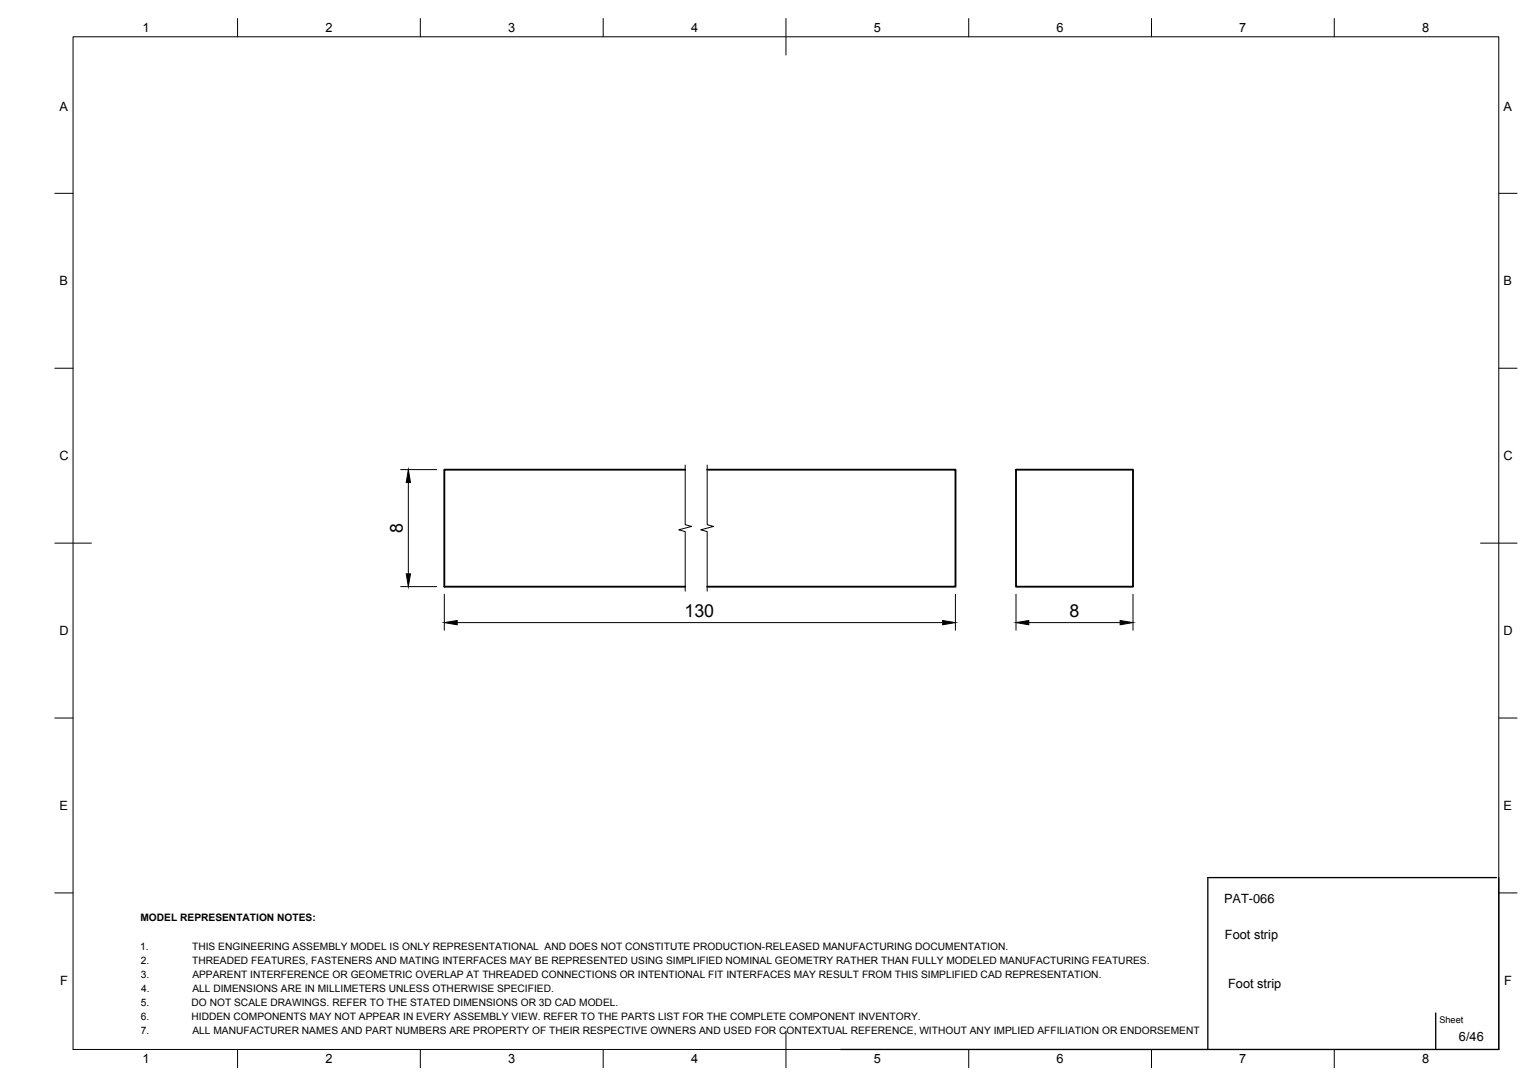
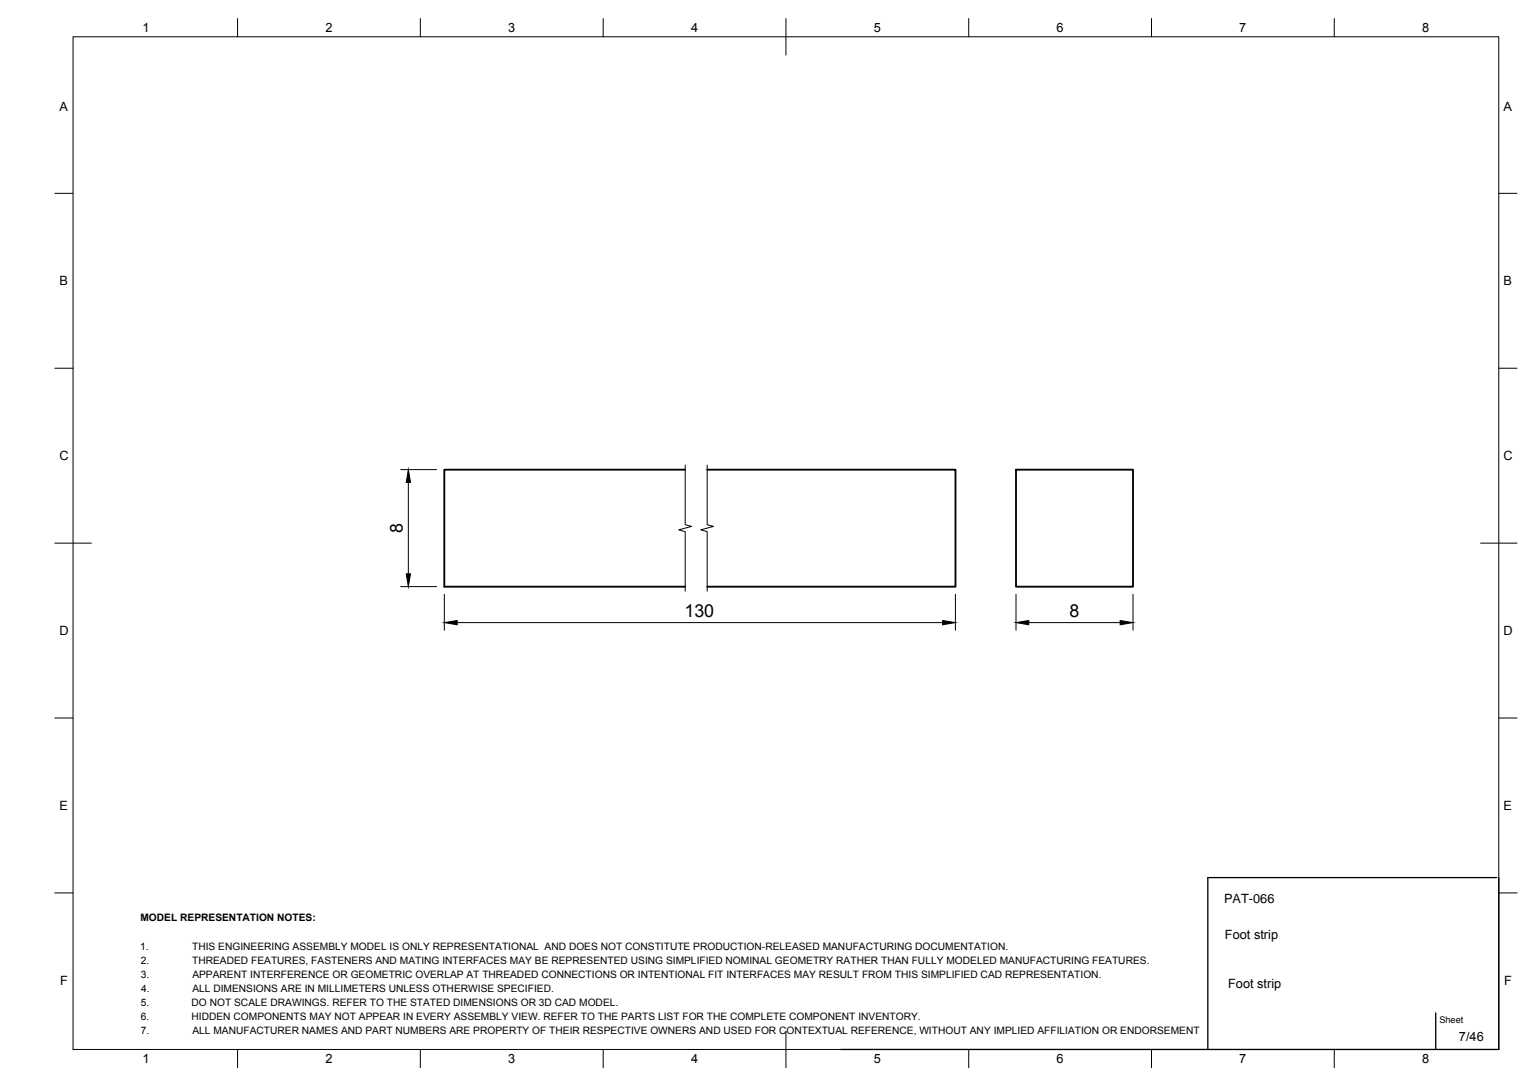
ISO-10303-21;
HEADER;
/* Generated by software containing ST-Developer
 * from STEP Tools, Inc. (www.steptools.com) 
 */

FILE_DESCRIPTION(
/* description */ ('Lever-operated bar clamp (toggle)'),
/* implementation_level */ '2;1');

FILE_NAME(
/* name */ 'Foot strip.step',
/* time_stamp */ '2026-10-28T03:25:02-07:00',
/* author */ (''),
/* organization */ (''),
/* preprocessor_version */ 'ST-DEVELOPER v20.2',
/* originating_system */ 'Autodesk Translation Framework v15.17.0.0',
/* authorisation */ '');

FILE_SCHEMA (('AUTOMOTIVE_DESIGN { 1 0 10303 214 3 1 1 }'));
ENDSEC;

DATA;
#10=MECHANICAL_DESIGN_GEOMETRIC_PRESENTATION_REPRESENTATION('',(#411),#12413);
#335=SHAPE_REPRESENTATION_RELATIONSHIP('SRR','None',#12574,#373);
#373=ADVANCED_BREP_SHAPE_REPRESENTATION('',(#458),#12371);
#411=STYLED_ITEM('',(#12855),#458);
#458=MANIFOLD_SOLID_BREP('Body1',#6570);
#657=PLANE('',#7073);
#658=PLANE('',#7074);
#659=PLANE('',#7075);
#660=PLANE('',#7076);
#661=PLANE('',#7077);
#662=PLANE('',#7078);
#902=FACE_OUTER_BOUND('',#1324,.T.);
#903=FACE_OUTER_BOUND('',#1325,.T.);
#904=FACE_OUTER_BOUND('',#1326,.T.);
#905=FACE_OUTER_BOUND('',#1327,.T.);
#906=FACE_OUTER_BOUND('',#1328,.T.);
#907=FACE_OUTER_BOUND('',#1329,.T.);
#1324=EDGE_LOOP('',(#4493,#4494,#4495,#4496));
#1325=EDGE_LOOP('',(#4497,#4498,#4499,#4500));
#1326=EDGE_LOOP('',(#4501,#4502,#4503,#4504));
#1327=EDGE_LOOP('',(#4505,#4506,#4507,#4508));
#1328=EDGE_LOOP('',(#4509,#4510,#4511,#4512));
#1329=EDGE_LOOP('',(#4513,#4514,#4515,#4516));
#1871=LINE('',#10126,#2312);
#1872=LINE('',#10128,#2313);
#1873=LINE('',#10130,#2314);
#1874=LINE('',#10131,#2315);
#1875=LINE('',#10134,#2316);
#1876=LINE('',#10136,#2317);
#1877=LINE('',#10137,#2318);
#1878=LINE('',#10140,#2319);
#1879=LINE('',#10142,#2320);
#1880=LINE('',#10143,#2321);
#1881=LINE('',#10145,#2322);
#1882=LINE('',#10146,#2323);
#2312=VECTOR('',#7984,1.);
#2313=VECTOR('',#7985,1.);
#2314=VECTOR('',#7986,1.);
#2315=VECTOR('',#7987,1.);
#2316=VECTOR('',#7990,1.);
#2317=VECTOR('',#7991,1.);
#2318=VECTOR('',#7992,1.);
#2319=VECTOR('',#7995,1.);
#2320=VECTOR('',#7996,1.);
#2321=VECTOR('',#7997,1.);
#2322=VECTOR('',#8000,1.);
#2323=VECTOR('',#8001,1.);
#3098=VERTEX_POINT('',#10124);
#3099=VERTEX_POINT('',#10125);
#3100=VERTEX_POINT('',#10127);
#3101=VERTEX_POINT('',#10129);
#3102=VERTEX_POINT('',#10133);
#3103=VERTEX_POINT('',#10135);
#3104=VERTEX_POINT('',#10139);
#3105=VERTEX_POINT('',#10141);
#3651=EDGE_CURVE('',#3098,#3099,#1871,.T.);
#3652=EDGE_CURVE('',#3099,#3100,#1872,.T.);
#3653=EDGE_CURVE('',#3101,#3100,#1873,.T.);
#3654=EDGE_CURVE('',#3098,#3101,#1874,.T.);
#3655=EDGE_CURVE('',#3102,#3098,#1875,.T.);
#3656=EDGE_CURVE('',#3103,#3101,#1876,.T.);
#3657=EDGE_CURVE('',#3102,#3103,#1877,.T.);
#3658=EDGE_CURVE('',#3104,#3102,#1878,.T.);
#3659=EDGE_CURVE('',#3105,#3103,#1879,.T.);
#3660=EDGE_CURVE('',#3104,#3105,#1880,.T.);
#3661=EDGE_CURVE('',#3099,#3104,#1881,.T.);
#3662=EDGE_CURVE('',#3100,#3105,#1882,.T.);
#4493=ORIENTED_EDGE('',*,*,#3651,.T.);
#4494=ORIENTED_EDGE('',*,*,#3652,.T.);
#4495=ORIENTED_EDGE('',*,*,#3653,.F.);
#4496=ORIENTED_EDGE('',*,*,#3654,.F.);
#4497=ORIENTED_EDGE('',*,*,#3655,.T.);
#4498=ORIENTED_EDGE('',*,*,#3654,.T.);
#4499=ORIENTED_EDGE('',*,*,#3656,.F.);
#4500=ORIENTED_EDGE('',*,*,#3657,.F.);
#4501=ORIENTED_EDGE('',*,*,#3658,.T.);
#4502=ORIENTED_EDGE('',*,*,#3657,.T.);
#4503=ORIENTED_EDGE('',*,*,#3659,.F.);
#4504=ORIENTED_EDGE('',*,*,#3660,.F.);
#4505=ORIENTED_EDGE('',*,*,#3661,.T.);
#4506=ORIENTED_EDGE('',*,*,#3660,.T.);
#4507=ORIENTED_EDGE('',*,*,#3662,.F.);
#4508=ORIENTED_EDGE('',*,*,#3652,.F.);
#4509=ORIENTED_EDGE('',*,*,#3662,.T.);
#4510=ORIENTED_EDGE('',*,*,#3659,.T.);
#4511=ORIENTED_EDGE('',*,*,#3656,.T.);
#4512=ORIENTED_EDGE('',*,*,#3653,.T.);
#4513=ORIENTED_EDGE('',*,*,#3661,.F.);
#4514=ORIENTED_EDGE('',*,*,#3651,.F.);
#4515=ORIENTED_EDGE('',*,*,#3655,.F.);
#4516=ORIENTED_EDGE('',*,*,#3658,.F.);
#6177=ADVANCED_FACE('',(#902),#657,.T.);
#6178=ADVANCED_FACE('',(#903),#658,.T.);
#6179=ADVANCED_FACE('',(#904),#659,.T.);
#6180=ADVANCED_FACE('',(#905),#660,.T.);
#6181=ADVANCED_FACE('',(#906),#661,.T.);
#6182=ADVANCED_FACE('',(#907),#662,.F.);
#6570=CLOSED_SHELL('',(#6177,#6178,#6179,#6180,#6181,#6182));
#7072=AXIS2_PLACEMENT_3D('',#10122,#7980,#7981);
#7073=AXIS2_PLACEMENT_3D('',#10123,#7982,#7983);
#7074=AXIS2_PLACEMENT_3D('',#10132,#7988,#7989);
#7075=AXIS2_PLACEMENT_3D('',#10138,#7993,#7994);
#7076=AXIS2_PLACEMENT_3D('',#10144,#7998,#7999);
#7077=AXIS2_PLACEMENT_3D('',#10147,#8002,#8003);
#7078=AXIS2_PLACEMENT_3D('',#10148,#8004,#8005);
#7980=DIRECTION('axis',(0.,0.,1.));
#7981=DIRECTION('refdir',(1.,0.,0.));
#7982=DIRECTION('center_axis',(0.,1.,0.));
#7983=DIRECTION('ref_axis',(-1.,0.,0.));
#7984=DIRECTION('',(-1.,0.,0.));
#7985=DIRECTION('',(0.,0.,1.));
#7986=DIRECTION('',(-1.,0.,0.));
#7987=DIRECTION('',(0.,0.,1.));
#7988=DIRECTION('center_axis',(1.,0.,0.));
#7989=DIRECTION('ref_axis',(0.,1.,0.));
#7990=DIRECTION('',(0.,1.,0.));
#7991=DIRECTION('',(0.,1.,0.));
#7992=DIRECTION('',(0.,0.,1.));
#7993=DIRECTION('center_axis',(0.,-1.,0.));
#7994=DIRECTION('ref_axis',(1.,0.,0.));
#7995=DIRECTION('',(1.,0.,0.));
#7996=DIRECTION('',(1.,0.,0.));
#7997=DIRECTION('',(0.,0.,1.));
#7998=DIRECTION('center_axis',(-1.,0.,0.));
#7999=DIRECTION('ref_axis',(0.,-1.,0.));
#8000=DIRECTION('',(0.,-1.,0.));
#8001=DIRECTION('',(0.,-1.,0.));
#8002=DIRECTION('center_axis',(0.,0.,1.));
#8003=DIRECTION('ref_axis',(1.,0.,0.));
#8004=DIRECTION('center_axis',(0.,0.,1.));
#8005=DIRECTION('ref_axis',(1.,0.,0.));
#10122=CARTESIAN_POINT('',(0.,0.,0.));
#10123=CARTESIAN_POINT('Origin',(3.5,-6.2,-0.8));
#10124=CARTESIAN_POINT('',(3.5,-6.2,-0.8));
#10125=CARTESIAN_POINT('',(-9.5,-6.2,-0.8));
#10126=CARTESIAN_POINT('',(3.5,-6.2,-0.8));
#10127=CARTESIAN_POINT('',(-9.5,-6.2,0.));
#10128=CARTESIAN_POINT('',(-9.5,-6.2,-0.8));
#10129=CARTESIAN_POINT('',(3.5,-6.2,0.));
#10130=CARTESIAN_POINT('',(3.5,-6.2,0.));
#10131=CARTESIAN_POINT('',(3.5,-6.2,-0.8));
#10132=CARTESIAN_POINT('Origin',(3.5,-7.,-0.8));
#10133=CARTESIAN_POINT('',(3.5,-7.,-0.8));
#10134=CARTESIAN_POINT('',(3.5,-7.,-0.8));
#10135=CARTESIAN_POINT('',(3.5,-7.,0.));
#10136=CARTESIAN_POINT('',(3.5,-7.,0.));
#10137=CARTESIAN_POINT('',(3.5,-7.,-0.8));
#10138=CARTESIAN_POINT('Origin',(-9.5,-7.,-0.8));
#10139=CARTESIAN_POINT('',(-9.5,-7.,-0.8));
#10140=CARTESIAN_POINT('',(-9.5,-7.,-0.8));
#10141=CARTESIAN_POINT('',(-9.5,-7.,0.));
#10142=CARTESIAN_POINT('',(-9.5,-7.,0.));
#10143=CARTESIAN_POINT('',(-9.5,-7.,-0.8));
#10144=CARTESIAN_POINT('Origin',(-9.5,-6.2,-0.8));
#10145=CARTESIAN_POINT('',(-9.5,-6.2,-0.8));
#10146=CARTESIAN_POINT('',(-9.5,-6.2,0.));
#10147=CARTESIAN_POINT('Origin',(-3.,-6.6,0.));
#10148=CARTESIAN_POINT('Origin',(-3.,-6.6,-0.8));
#12325=UNCERTAINTY_MEASURE_WITH_UNIT(LENGTH_MEASURE(0.001),#12414,
'DISTANCE_ACCURACY_VALUE',
'Maximum model space distance between geometric entities at asserted c
onnectivities');
#12367=UNCERTAINTY_MEASURE_WITH_UNIT(LENGTH_MEASURE(0.001),#12414,
'DISTANCE_ACCURACY_VALUE',
'Maximum model space distance between geometric entities at asserted c
onnectivities');
#12371=(
GEOMETRIC_REPRESENTATION_CONTEXT(3)
GLOBAL_UNCERTAINTY_ASSIGNED_CONTEXT((#12325))
GLOBAL_UNIT_ASSIGNED_CONTEXT((#12414,#12416,#12417))
REPRESENTATION_CONTEXT('','3D')
);
#12413=(
GEOMETRIC_REPRESENTATION_CONTEXT(3)
GLOBAL_UNCERTAINTY_ASSIGNED_CONTEXT((#12367))
GLOBAL_UNIT_ASSIGNED_CONTEXT((#12414,#12416,#12417))
REPRESENTATION_CONTEXT('','3D')
);
#12414=(
LENGTH_UNIT()
NAMED_UNIT(*)
SI_UNIT(.CENTI.,.METRE.)
);
#12416=(
NAMED_UNIT(*)
PLANE_ANGLE_UNIT()
SI_UNIT($,.RADIAN.)
);
#12417=(
NAMED_UNIT(*)
SI_UNIT($,.STERADIAN.)
SOLID_ANGLE_UNIT()
);
#12421=SHAPE_DEFINITION_REPRESENTATION(#12466,#12574);
#12466=PRODUCT_DEFINITION_SHAPE('',$,#12620);
#12574=SHAPE_REPRESENTATION('',(#7072),#12371);
#12616=PRODUCT_DEFINITION_CONTEXT('part definition',#12753,'design');
#12620=PRODUCT_DEFINITION('Foot strip','Foot strip',#12665,#12616);
#12665=PRODUCT_DEFINITION_FORMATION('',$,#12758);
#12753=APPLICATION_CONTEXT(
'Core Data for Automotive Mechanical Design Process');
#12754=PRODUCT_CONTEXT('part definition',#12753,'mechanical');
#12758=PRODUCT('Foot strip','Foot strip','Foot strip',(#12754));
#12849=COLOUR_RGB('Light Blue',0.38,0.62,0.78);
#12850=FILL_AREA_STYLE_COLOUR('',#12849);
#12851=FILL_AREA_STYLE('',(#12850));
#12852=SURFACE_STYLE_FILL_AREA(#12851);
#12853=SURFACE_SIDE_STYLE('',(#12852));
#12854=SURFACE_STYLE_USAGE(.BOTH.,#12853);
#12855=PRESENTATION_STYLE_ASSIGNMENT((#12854));
ENDSEC;
END-ISO-10303-21;
